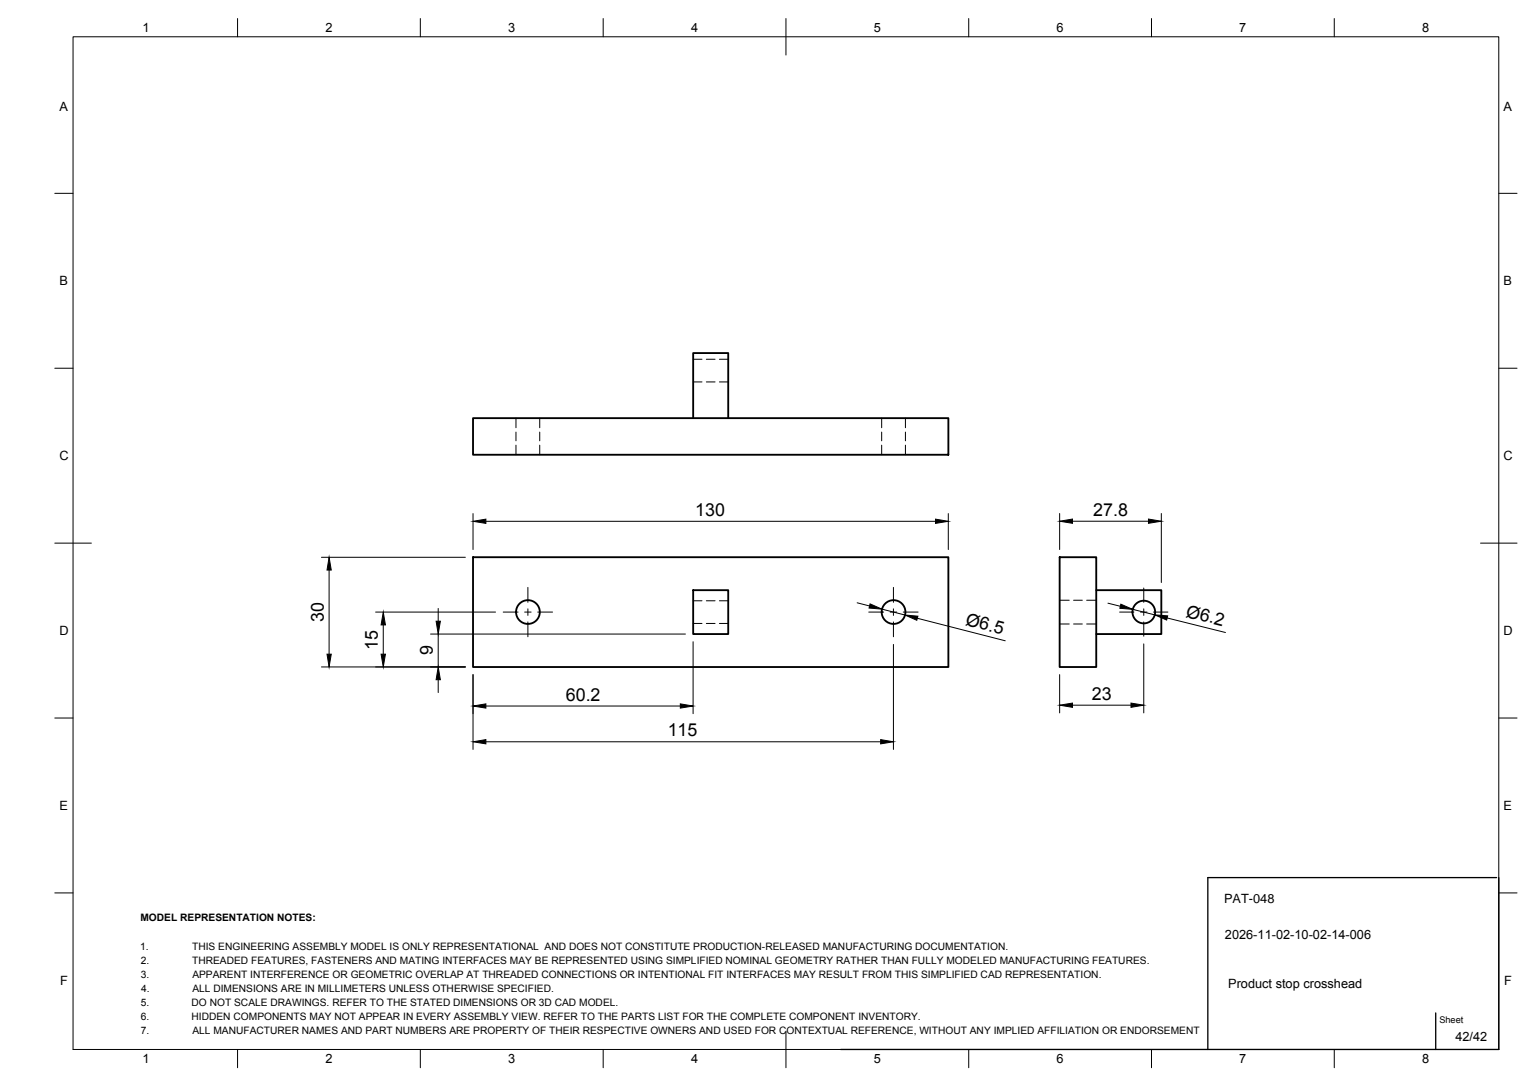
ISO-10303-21;
HEADER;
/* Generated by software containing ST-Developer
 * from STEP Tools, Inc. (www.steptools.com) 
 */

FILE_DESCRIPTION(
/* description */ ('Guided pneumatic stop gate'),
/* implementation_level */ '2;1');

FILE_NAME(
/* name */ 'Product stop crosshead.step',
/* time_stamp */ '2026-10-27T21:43:45-07:00',
/* author */ (''),
/* organization */ (''),
/* preprocessor_version */ 'ST-DEVELOPER v20.2',
/* originating_system */ 'Autodesk Translation Framework v15.17.0.0',
/* authorisation */ '');

FILE_SCHEMA (('AUTOMOTIVE_DESIGN { 1 0 10303 214 3 1 1 }'));
ENDSEC;

DATA;
#10=MECHANICAL_DESIGN_GEOMETRIC_PRESENTATION_REPRESENTATION('',(#574),#14392);
#490=SHAPE_REPRESENTATION_RELATIONSHIP('SRR','None',#14627,#532);
#532=ADVANCED_BREP_SHAPE_REPRESENTATION('',(#612),#14389);
#574=STYLED_ITEM('',(#14891),#612);
#612=MANIFOLD_SOLID_BREP('Body1',#7918);
#814=FACE_BOUND('',#2243,.T.);
#815=FACE_BOUND('',#2246,.T.);
#816=FACE_BOUND('',#2249,.T.);
#817=FACE_BOUND('',#2250,.T.);
#818=FACE_BOUND('',#2251,.T.);
#819=FACE_BOUND('',#2254,.T.);
#820=FACE_BOUND('',#2255,.T.);
#1097=PLANE('',#9325);
#1098=PLANE('',#9326);
#1099=PLANE('',#9327);
#1100=PLANE('',#9328);
#1101=PLANE('',#9329);
#1102=PLANE('',#9330);
#1103=PLANE('',#9331);
#1104=PLANE('',#9332);
#1105=PLANE('',#9333);
#1106=PLANE('',#9334);
#1107=PLANE('',#9335);
#1564=FACE_OUTER_BOUND('',#2238,.T.);
#1565=FACE_OUTER_BOUND('',#2239,.T.);
#1566=FACE_OUTER_BOUND('',#2240,.T.);
#1567=FACE_OUTER_BOUND('',#2241,.T.);
#1568=FACE_OUTER_BOUND('',#2242,.T.);
#1569=FACE_OUTER_BOUND('',#2244,.T.);
#1570=FACE_OUTER_BOUND('',#2245,.T.);
#1571=FACE_OUTER_BOUND('',#2247,.T.);
#1572=FACE_OUTER_BOUND('',#2248,.T.);
#1573=FACE_OUTER_BOUND('',#2252,.T.);
#1574=FACE_OUTER_BOUND('',#2253,.T.);
#1575=FACE_OUTER_BOUND('',#2256,.T.);
#1576=FACE_OUTER_BOUND('',#2257,.T.);
#1577=FACE_OUTER_BOUND('',#2258,.T.);
#2238=EDGE_LOOP('',(#7108,#7109,#7110,#7111));
#2239=EDGE_LOOP('',(#7112,#7113,#7114,#7115));
#2240=EDGE_LOOP('',(#7116,#7117,#7118,#7119));
#2241=EDGE_LOOP('',(#7120,#7121,#7122,#7123));
#2242=EDGE_LOOP('',(#7124,#7125,#7126,#7127));
#2243=EDGE_LOOP('',(#7128));
#2244=EDGE_LOOP('',(#7129,#7130,#7131,#7132));
#2245=EDGE_LOOP('',(#7133,#7134,#7135,#7136));
#2246=EDGE_LOOP('',(#7137));
#2247=EDGE_LOOP('',(#7138,#7139,#7140,#7141));
#2248=EDGE_LOOP('',(#7142,#7143,#7144,#7145));
#2249=EDGE_LOOP('',(#7146));
#2250=EDGE_LOOP('',(#7147));
#2251=EDGE_LOOP('',(#7148,#7149,#7150,#7151));
#2252=EDGE_LOOP('',(#7152,#7153,#7154,#7155));
#2253=EDGE_LOOP('',(#7156,#7157,#7158,#7159));
#2254=EDGE_LOOP('',(#7160));
#2255=EDGE_LOOP('',(#7161));
#2256=EDGE_LOOP('',(#7162,#7163,#7164,#7165));
#2257=EDGE_LOOP('',(#7166,#7167,#7168,#7169));
#2258=EDGE_LOOP('',(#7170,#7171,#7172,#7173));
#2785=LINE('',#14120,#3330);
#2786=LINE('',#14126,#3331);
#2787=LINE('',#14132,#3332);
#2788=LINE('',#14137,#3333);
#2789=LINE('',#14139,#3334);
#2790=LINE('',#14141,#3335);
#2791=LINE('',#14142,#3336);
#2792=LINE('',#14145,#3337);
#2793=LINE('',#14147,#3338);
#2794=LINE('',#14148,#3339);
#2795=LINE('',#14151,#3340);
#2796=LINE('',#14152,#3341);
#2797=LINE('',#14155,#3342);
#2798=LINE('',#14156,#3343);
#2799=LINE('',#14158,#3344);
#2800=LINE('',#14162,#3345);
#2801=LINE('',#14164,#3346);
#2802=LINE('',#14166,#3347);
#2803=LINE('',#14167,#3348);
#2804=LINE('',#14170,#3349);
#2805=LINE('',#14172,#3350);
#2806=LINE('',#14173,#3351);
#2807=LINE('',#14176,#3352);
#2808=LINE('',#14178,#3353);
#2809=LINE('',#14179,#3354);
#2810=LINE('',#14181,#3355);
#2811=LINE('',#14182,#3356);
#3330=VECTOR('',#11756,0.325);
#3331=VECTOR('',#11763,0.325);
#3332=VECTOR('',#11770,0.31);
#3333=VECTOR('',#11775,1.);
#3334=VECTOR('',#11776,1.);
#3335=VECTOR('',#11777,1.);
#3336=VECTOR('',#11778,1.);
#3337=VECTOR('',#11781,1.);
#3338=VECTOR('',#11782,1.);
#3339=VECTOR('',#11783,1.);
#3340=VECTOR('',#11786,1.);
#3341=VECTOR('',#11787,1.);
#3342=VECTOR('',#11790,1.);
#3343=VECTOR('',#11791,1.);
#3344=VECTOR('',#11794,1.);
#3345=VECTOR('',#11797,1.);
#3346=VECTOR('',#11798,1.);
#3347=VECTOR('',#11799,1.);
#3348=VECTOR('',#11800,1.);
#3349=VECTOR('',#11803,1.);
#3350=VECTOR('',#11804,1.);
#3351=VECTOR('',#11805,1.);
#3352=VECTOR('',#11808,1.);
#3353=VECTOR('',#11809,1.);
#3354=VECTOR('',#11810,1.);
#3355=VECTOR('',#11813,1.);
#3356=VECTOR('',#11814,1.);
#3723=CIRCLE('',#9317,0.325);
#3724=CIRCLE('',#9318,0.325);
#3725=CIRCLE('',#9320,0.325);
#3726=CIRCLE('',#9321,0.325);
#3727=CIRCLE('',#9323,0.31);
#3728=CIRCLE('',#9324,0.31);
#4314=VERTEX_POINT('',#14117);
#4315=VERTEX_POINT('',#14119);
#4316=VERTEX_POINT('',#14123);
#4317=VERTEX_POINT('',#14125);
#4318=VERTEX_POINT('',#14129);
#4319=VERTEX_POINT('',#14131);
#4320=VERTEX_POINT('',#14135);
#4321=VERTEX_POINT('',#14136);
#4322=VERTEX_POINT('',#14138);
#4323=VERTEX_POINT('',#14140);
#4324=VERTEX_POINT('',#14144);
#4325=VERTEX_POINT('',#14146);
#4326=VERTEX_POINT('',#14150);
#4327=VERTEX_POINT('',#14154);
#4328=VERTEX_POINT('',#14160);
#4329=VERTEX_POINT('',#14161);
#4330=VERTEX_POINT('',#14163);
#4331=VERTEX_POINT('',#14165);
#4332=VERTEX_POINT('',#14169);
#4333=VERTEX_POINT('',#14171);
#4334=VERTEX_POINT('',#14175);
#4335=VERTEX_POINT('',#14177);
#5252=EDGE_CURVE('',#4314,#4314,#3723,.T.);
#5253=EDGE_CURVE('',#4314,#4315,#2785,.T.);
#5254=EDGE_CURVE('',#4315,#4315,#3724,.T.);
#5255=EDGE_CURVE('',#4316,#4316,#3725,.T.);
#5256=EDGE_CURVE('',#4316,#4317,#2786,.T.);
#5257=EDGE_CURVE('',#4317,#4317,#3726,.T.);
#5258=EDGE_CURVE('',#4318,#4318,#3727,.T.);
#5259=EDGE_CURVE('',#4318,#4319,#2787,.T.);
#5260=EDGE_CURVE('',#4319,#4319,#3728,.T.);
#5261=EDGE_CURVE('',#4320,#4321,#2788,.T.);
#5262=EDGE_CURVE('',#4322,#4320,#2789,.T.);
#5263=EDGE_CURVE('',#4323,#4322,#2790,.T.);
#5264=EDGE_CURVE('',#4321,#4323,#2791,.T.);
#5265=EDGE_CURVE('',#4324,#4320,#2792,.T.);
#5266=EDGE_CURVE('',#4325,#4324,#2793,.T.);
#5267=EDGE_CURVE('',#4322,#4325,#2794,.T.);
#5268=EDGE_CURVE('',#4326,#4325,#2795,.T.);
#5269=EDGE_CURVE('',#4323,#4326,#2796,.T.);
#5270=EDGE_CURVE('',#4321,#4327,#2797,.T.);
#5271=EDGE_CURVE('',#4327,#4326,#2798,.T.);
#5272=EDGE_CURVE('',#4327,#4324,#2799,.T.);
#5273=EDGE_CURVE('',#4328,#4329,#2800,.T.);
#5274=EDGE_CURVE('',#4329,#4330,#2801,.T.);
#5275=EDGE_CURVE('',#4331,#4330,#2802,.T.);
#5276=EDGE_CURVE('',#4328,#4331,#2803,.T.);
#5277=EDGE_CURVE('',#4332,#4328,#2804,.T.);
#5278=EDGE_CURVE('',#4333,#4331,#2805,.T.);
#5279=EDGE_CURVE('',#4332,#4333,#2806,.T.);
#5280=EDGE_CURVE('',#4334,#4332,#2807,.T.);
#5281=EDGE_CURVE('',#4335,#4333,#2808,.T.);
#5282=EDGE_CURVE('',#4334,#4335,#2809,.T.);
#5283=EDGE_CURVE('',#4329,#4334,#2810,.T.);
#5284=EDGE_CURVE('',#4330,#4335,#2811,.T.);
#7108=ORIENTED_EDGE('',*,*,#5252,.F.);
#7109=ORIENTED_EDGE('',*,*,#5253,.T.);
#7110=ORIENTED_EDGE('',*,*,#5254,.F.);
#7111=ORIENTED_EDGE('',*,*,#5253,.F.);
#7112=ORIENTED_EDGE('',*,*,#5255,.F.);
#7113=ORIENTED_EDGE('',*,*,#5256,.T.);
#7114=ORIENTED_EDGE('',*,*,#5257,.F.);
#7115=ORIENTED_EDGE('',*,*,#5256,.F.);
#7116=ORIENTED_EDGE('',*,*,#5258,.F.);
#7117=ORIENTED_EDGE('',*,*,#5259,.T.);
#7118=ORIENTED_EDGE('',*,*,#5260,.F.);
#7119=ORIENTED_EDGE('',*,*,#5259,.F.);
#7120=ORIENTED_EDGE('',*,*,#5261,.F.);
#7121=ORIENTED_EDGE('',*,*,#5262,.F.);
#7122=ORIENTED_EDGE('',*,*,#5263,.F.);
#7123=ORIENTED_EDGE('',*,*,#5264,.F.);
#7124=ORIENTED_EDGE('',*,*,#5265,.F.);
#7125=ORIENTED_EDGE('',*,*,#5266,.F.);
#7126=ORIENTED_EDGE('',*,*,#5267,.F.);
#7127=ORIENTED_EDGE('',*,*,#5262,.T.);
#7128=ORIENTED_EDGE('',*,*,#5258,.T.);
#7129=ORIENTED_EDGE('',*,*,#5263,.T.);
#7130=ORIENTED_EDGE('',*,*,#5267,.T.);
#7131=ORIENTED_EDGE('',*,*,#5268,.F.);
#7132=ORIENTED_EDGE('',*,*,#5269,.F.);
#7133=ORIENTED_EDGE('',*,*,#5270,.F.);
#7134=ORIENTED_EDGE('',*,*,#5264,.T.);
#7135=ORIENTED_EDGE('',*,*,#5269,.T.);
#7136=ORIENTED_EDGE('',*,*,#5271,.F.);
#7137=ORIENTED_EDGE('',*,*,#5260,.T.);
#7138=ORIENTED_EDGE('',*,*,#5272,.F.);
#7139=ORIENTED_EDGE('',*,*,#5271,.T.);
#7140=ORIENTED_EDGE('',*,*,#5268,.T.);
#7141=ORIENTED_EDGE('',*,*,#5266,.T.);
#7142=ORIENTED_EDGE('',*,*,#5273,.T.);
#7143=ORIENTED_EDGE('',*,*,#5274,.T.);
#7144=ORIENTED_EDGE('',*,*,#5275,.F.);
#7145=ORIENTED_EDGE('',*,*,#5276,.F.);
#7146=ORIENTED_EDGE('',*,*,#5254,.T.);
#7147=ORIENTED_EDGE('',*,*,#5257,.T.);
#7148=ORIENTED_EDGE('',*,*,#5265,.T.);
#7149=ORIENTED_EDGE('',*,*,#5261,.T.);
#7150=ORIENTED_EDGE('',*,*,#5270,.T.);
#7151=ORIENTED_EDGE('',*,*,#5272,.T.);
#7152=ORIENTED_EDGE('',*,*,#5277,.T.);
#7153=ORIENTED_EDGE('',*,*,#5276,.T.);
#7154=ORIENTED_EDGE('',*,*,#5278,.F.);
#7155=ORIENTED_EDGE('',*,*,#5279,.F.);
#7156=ORIENTED_EDGE('',*,*,#5280,.T.);
#7157=ORIENTED_EDGE('',*,*,#5279,.T.);
#7158=ORIENTED_EDGE('',*,*,#5281,.F.);
#7159=ORIENTED_EDGE('',*,*,#5282,.F.);
#7160=ORIENTED_EDGE('',*,*,#5252,.T.);
#7161=ORIENTED_EDGE('',*,*,#5255,.T.);
#7162=ORIENTED_EDGE('',*,*,#5283,.T.);
#7163=ORIENTED_EDGE('',*,*,#5282,.T.);
#7164=ORIENTED_EDGE('',*,*,#5284,.F.);
#7165=ORIENTED_EDGE('',*,*,#5274,.F.);
#7166=ORIENTED_EDGE('',*,*,#5284,.T.);
#7167=ORIENTED_EDGE('',*,*,#5281,.T.);
#7168=ORIENTED_EDGE('',*,*,#5278,.T.);
#7169=ORIENTED_EDGE('',*,*,#5275,.T.);
#7170=ORIENTED_EDGE('',*,*,#5283,.F.);
#7171=ORIENTED_EDGE('',*,*,#5273,.F.);
#7172=ORIENTED_EDGE('',*,*,#5277,.F.);
#7173=ORIENTED_EDGE('',*,*,#5280,.F.);
#7394=CYLINDRICAL_SURFACE('',#9316,0.325);
#7395=CYLINDRICAL_SURFACE('',#9319,0.325);
#7396=CYLINDRICAL_SURFACE('',#9322,0.31);
#7846=ADVANCED_FACE('',(#1564),#7394,.F.);
#7847=ADVANCED_FACE('',(#1565),#7395,.F.);
#7848=ADVANCED_FACE('',(#1566),#7396,.F.);
#7849=ADVANCED_FACE('',(#1567),#1097,.F.);
#7850=ADVANCED_FACE('',(#1568,#814),#1098,.T.);
#7851=ADVANCED_FACE('',(#1569),#1099,.T.);
#7852=ADVANCED_FACE('',(#1570,#815),#1100,.T.);
#7853=ADVANCED_FACE('',(#1571),#1101,.T.);
#7854=ADVANCED_FACE('',(#1572,#816,#817,#818),#1102,.T.);
#7855=ADVANCED_FACE('',(#1573),#1103,.T.);
#7856=ADVANCED_FACE('',(#1574,#819,#820),#1104,.T.);
#7857=ADVANCED_FACE('',(#1575),#1105,.T.);
#7858=ADVANCED_FACE('',(#1576),#1106,.T.);
#7859=ADVANCED_FACE('',(#1577),#1107,.F.);
#7918=CLOSED_SHELL('',(#7846,#7847,#7848,#7849,#7850,#7851,#7852,#7853,
#7854,#7855,#7856,#7857,#7858,#7859));
#9315=AXIS2_PLACEMENT_3D('',#14115,#11750,#11751);
#9316=AXIS2_PLACEMENT_3D('',#14116,#11752,#11753);
#9317=AXIS2_PLACEMENT_3D('',#14118,#11754,#11755);
#9318=AXIS2_PLACEMENT_3D('',#14121,#11757,#11758);
#9319=AXIS2_PLACEMENT_3D('',#14122,#11759,#11760);
#9320=AXIS2_PLACEMENT_3D('',#14124,#11761,#11762);
#9321=AXIS2_PLACEMENT_3D('',#14127,#11764,#11765);
#9322=AXIS2_PLACEMENT_3D('',#14128,#11766,#11767);
#9323=AXIS2_PLACEMENT_3D('',#14130,#11768,#11769);
#9324=AXIS2_PLACEMENT_3D('',#14133,#11771,#11772);
#9325=AXIS2_PLACEMENT_3D('',#14134,#11773,#11774);
#9326=AXIS2_PLACEMENT_3D('',#14143,#11779,#11780);
#9327=AXIS2_PLACEMENT_3D('',#14149,#11784,#11785);
#9328=AXIS2_PLACEMENT_3D('',#14153,#11788,#11789);
#9329=AXIS2_PLACEMENT_3D('',#14157,#11792,#11793);
#9330=AXIS2_PLACEMENT_3D('',#14159,#11795,#11796);
#9331=AXIS2_PLACEMENT_3D('',#14168,#11801,#11802);
#9332=AXIS2_PLACEMENT_3D('',#14174,#11806,#11807);
#9333=AXIS2_PLACEMENT_3D('',#14180,#11811,#11812);
#9334=AXIS2_PLACEMENT_3D('',#14183,#11815,#11816);
#9335=AXIS2_PLACEMENT_3D('',#14184,#11817,#11818);
#11750=DIRECTION('axis',(0.,0.,1.));
#11751=DIRECTION('refdir',(1.,0.,0.));
#11752=DIRECTION('center_axis',(0.,1.,0.));
#11753=DIRECTION('ref_axis',(1.,0.,0.));
#11754=DIRECTION('center_axis',(0.,1.,0.));
#11755=DIRECTION('ref_axis',(1.,0.,0.));
#11756=DIRECTION('',(0.,1.,0.));
#11757=DIRECTION('center_axis',(0.,-1.,0.));
#11758=DIRECTION('ref_axis',(1.,0.,0.));
#11759=DIRECTION('center_axis',(0.,1.,0.));
#11760=DIRECTION('ref_axis',(1.,0.,0.));
#11761=DIRECTION('center_axis',(0.,1.,0.));
#11762=DIRECTION('ref_axis',(1.,0.,0.));
#11763=DIRECTION('',(0.,1.,0.));
#11764=DIRECTION('center_axis',(0.,-1.,0.));
#11765=DIRECTION('ref_axis',(1.,0.,0.));
#11766=DIRECTION('center_axis',(1.,0.,0.));
#11767=DIRECTION('ref_axis',(0.,0.,-1.));
#11768=DIRECTION('center_axis',(1.,0.,0.));
#11769=DIRECTION('ref_axis',(0.,0.,-1.));
#11770=DIRECTION('',(1.,0.,0.));
#11771=DIRECTION('center_axis',(-1.,0.,0.));
#11772=DIRECTION('ref_axis',(0.,0.,-1.));
#11773=DIRECTION('center_axis',(0.,0.,1.));
#11774=DIRECTION('ref_axis',(1.,0.,0.));
#11775=DIRECTION('',(1.,0.,0.));
#11776=DIRECTION('',(0.,-1.,0.));
#11777=DIRECTION('',(-1.,0.,0.));
#11778=DIRECTION('',(0.,1.,0.));
#11779=DIRECTION('center_axis',(-1.,0.,0.));
#11780=DIRECTION('ref_axis',(0.,-1.,0.));
#11781=DIRECTION('',(0.,0.,-1.));
#11782=DIRECTION('',(0.,-1.,0.));
#11783=DIRECTION('',(0.,0.,1.));
#11784=DIRECTION('center_axis',(0.,1.,0.));
#11785=DIRECTION('ref_axis',(-1.,0.,0.));
#11786=DIRECTION('',(-1.,0.,0.));
#11787=DIRECTION('',(0.,0.,1.));
#11788=DIRECTION('center_axis',(1.,0.,0.));
#11789=DIRECTION('ref_axis',(0.,1.,0.));
#11790=DIRECTION('',(0.,0.,1.));
#11791=DIRECTION('',(0.,1.,0.));
#11792=DIRECTION('center_axis',(0.,0.,1.));
#11793=DIRECTION('ref_axis',(1.,0.,0.));
#11794=DIRECTION('',(-1.,0.,0.));
#11795=DIRECTION('center_axis',(0.,1.,0.));
#11796=DIRECTION('ref_axis',(-1.,0.,0.));
#11797=DIRECTION('',(-1.,0.,0.));
#11798=DIRECTION('',(0.,0.,1.));
#11799=DIRECTION('',(-1.,0.,0.));
#11800=DIRECTION('',(0.,0.,1.));
#11801=DIRECTION('center_axis',(1.,0.,0.));
#11802=DIRECTION('ref_axis',(0.,1.,0.));
#11803=DIRECTION('',(0.,1.,0.));
#11804=DIRECTION('',(0.,1.,0.));
#11805=DIRECTION('',(0.,0.,1.));
#11806=DIRECTION('center_axis',(0.,-1.,0.));
#11807=DIRECTION('ref_axis',(1.,0.,0.));
#11808=DIRECTION('',(1.,0.,0.));
#11809=DIRECTION('',(1.,0.,0.));
#11810=DIRECTION('',(0.,0.,1.));
#11811=DIRECTION('center_axis',(-1.,0.,0.));
#11812=DIRECTION('ref_axis',(0.,-1.,0.));
#11813=DIRECTION('',(0.,-1.,0.));
#11814=DIRECTION('',(0.,-1.,0.));
#11815=DIRECTION('center_axis',(0.,0.,1.));
#11816=DIRECTION('ref_axis',(1.,0.,0.));
#11817=DIRECTION('center_axis',(0.,0.,1.));
#11818=DIRECTION('ref_axis',(1.,0.,0.));
#14115=CARTESIAN_POINT('',(0.,0.,0.));
#14116=CARTESIAN_POINT('Origin',(-5.,-8.5,4.5));
#14117=CARTESIAN_POINT('',(-5.325,-8.4,4.5));
#14118=CARTESIAN_POINT('Origin',(-5.,-8.4,4.5));
#14119=CARTESIAN_POINT('',(-5.325,-7.4,4.5));
#14120=CARTESIAN_POINT('',(-5.325,-8.5,4.5));
#14121=CARTESIAN_POINT('Origin',(-5.,-7.4,4.5));
#14122=CARTESIAN_POINT('Origin',(5.,-8.5,4.5));
#14123=CARTESIAN_POINT('',(4.675,-8.4,4.5));
#14124=CARTESIAN_POINT('Origin',(5.,-8.4,4.5));
#14125=CARTESIAN_POINT('',(4.675,-7.4,4.5));
#14126=CARTESIAN_POINT('',(4.675,-8.5,4.5));
#14127=CARTESIAN_POINT('Origin',(5.,-7.4,4.5));
#14128=CARTESIAN_POINT('Origin',(-0.6,-6.1,4.5));
#14129=CARTESIAN_POINT('',(-0.48,-6.1,4.81));
#14130=CARTESIAN_POINT('Origin',(-0.48,-6.1,4.5));
#14131=CARTESIAN_POINT('',(0.48,-6.1,4.81));
#14132=CARTESIAN_POINT('',(-0.6,-6.1,4.81));
#14133=CARTESIAN_POINT('Origin',(0.48,-6.1,4.5));
#14134=CARTESIAN_POINT('Origin',(0.,-7.01,3.9));
#14135=CARTESIAN_POINT('',(-0.48,-7.4,3.9));
#14136=CARTESIAN_POINT('',(0.48,-7.4,3.9));
#14137=CARTESIAN_POINT('',(3.25,-7.4,3.9));
#14138=CARTESIAN_POINT('',(-0.48,-5.62,3.9));
#14139=CARTESIAN_POINT('',(-0.48,-5.62,3.9));
#14140=CARTESIAN_POINT('',(0.48,-5.62,3.9));
#14141=CARTESIAN_POINT('',(0.48,-5.62,3.9));
#14142=CARTESIAN_POINT('',(0.48,-8.4,3.9));
#14143=CARTESIAN_POINT('Origin',(-0.48,-5.62,3.9));
#14144=CARTESIAN_POINT('',(-0.48,-7.4,5.1));
#14145=CARTESIAN_POINT('',(-0.48,-7.4,3.45));
#14146=CARTESIAN_POINT('',(-0.48,-5.62,5.1));
#14147=CARTESIAN_POINT('',(-0.48,-5.62,5.1));
#14148=CARTESIAN_POINT('',(-0.48,-5.62,3.9));
#14149=CARTESIAN_POINT('Origin',(0.48,-5.62,3.9));
#14150=CARTESIAN_POINT('',(0.48,-5.62,5.1));
#14151=CARTESIAN_POINT('',(0.48,-5.62,5.1));
#14152=CARTESIAN_POINT('',(0.48,-5.62,3.9));
#14153=CARTESIAN_POINT('Origin',(0.48,-8.4,3.9));
#14154=CARTESIAN_POINT('',(0.48,-7.4,5.1));
#14155=CARTESIAN_POINT('',(0.48,-7.4,3.45));
#14156=CARTESIAN_POINT('',(0.48,-8.4,5.1));
#14157=CARTESIAN_POINT('Origin',(0.,-7.01,5.1));
#14158=CARTESIAN_POINT('',(3.25,-7.4,5.1));
#14159=CARTESIAN_POINT('Origin',(6.5,-7.4,3.));
#14160=CARTESIAN_POINT('',(6.5,-7.4,3.));
#14161=CARTESIAN_POINT('',(-6.5,-7.4,3.));
#14162=CARTESIAN_POINT('',(6.5,-7.4,3.));
#14163=CARTESIAN_POINT('',(-6.5,-7.4,6.));
#14164=CARTESIAN_POINT('',(-6.5,-7.4,3.));
#14165=CARTESIAN_POINT('',(6.5,-7.4,6.));
#14166=CARTESIAN_POINT('',(6.5,-7.4,6.));
#14167=CARTESIAN_POINT('',(6.5,-7.4,3.));
#14168=CARTESIAN_POINT('Origin',(6.5,-8.4,3.));
#14169=CARTESIAN_POINT('',(6.5,-8.4,3.));
#14170=CARTESIAN_POINT('',(6.5,-8.4,3.));
#14171=CARTESIAN_POINT('',(6.5,-8.4,6.));
#14172=CARTESIAN_POINT('',(6.5,-8.4,6.));
#14173=CARTESIAN_POINT('',(6.5,-8.4,3.));
#14174=CARTESIAN_POINT('Origin',(-6.5,-8.4,3.));
#14175=CARTESIAN_POINT('',(-6.5,-8.4,3.));
#14176=CARTESIAN_POINT('',(-6.5,-8.4,3.));
#14177=CARTESIAN_POINT('',(-6.5,-8.4,6.));
#14178=CARTESIAN_POINT('',(-6.5,-8.4,6.));
#14179=CARTESIAN_POINT('',(-6.5,-8.4,3.));
#14180=CARTESIAN_POINT('Origin',(-6.5,-7.4,3.));
#14181=CARTESIAN_POINT('',(-6.5,-7.4,3.));
#14182=CARTESIAN_POINT('',(-6.5,-7.4,6.));
#14183=CARTESIAN_POINT('Origin',(0.,-7.9,6.));
#14184=CARTESIAN_POINT('Origin',(0.,-7.9,3.));
#14341=UNCERTAINTY_MEASURE_WITH_UNIT(LENGTH_MEASURE(0.001),#14393,
'DISTANCE_ACCURACY_VALUE',
'Maximum model space distance between geometric entities at asserted c
onnectivities');
#14344=UNCERTAINTY_MEASURE_WITH_UNIT(LENGTH_MEASURE(0.001),#14393,
'DISTANCE_ACCURACY_VALUE',
'Maximum model space distance between geometric entities at asserted c
onnectivities');
#14389=(
GEOMETRIC_REPRESENTATION_CONTEXT(3)
GLOBAL_UNCERTAINTY_ASSIGNED_CONTEXT((#14341))
GLOBAL_UNIT_ASSIGNED_CONTEXT((#14393,#14395,#14396))
REPRESENTATION_CONTEXT('','3D')
);
#14392=(
GEOMETRIC_REPRESENTATION_CONTEXT(3)
GLOBAL_UNCERTAINTY_ASSIGNED_CONTEXT((#14344))
GLOBAL_UNIT_ASSIGNED_CONTEXT((#14393,#14395,#14396))
REPRESENTATION_CONTEXT('','3D')
);
#14393=(
LENGTH_UNIT()
NAMED_UNIT(*)
SI_UNIT(.CENTI.,.METRE.)
);
#14395=(
NAMED_UNIT(*)
PLANE_ANGLE_UNIT()
SI_UNIT($,.RADIAN.)
);
#14396=(
NAMED_UNIT(*)
SI_UNIT($,.STERADIAN.)
SOLID_ANGLE_UNIT()
);
#14441=SHAPE_DEFINITION_REPRESENTATION(#14560,#14627);
#14560=PRODUCT_DEFINITION_SHAPE('',$,#14675);
#14627=SHAPE_REPRESENTATION('',(#9315),#14389);
#14630=PRODUCT_DEFINITION_CONTEXT('part definition',#14773,'design');
#14675=PRODUCT_DEFINITION('Product stop crosshead',
'Product stop crosshead',#14722,#14630);
#14722=PRODUCT_DEFINITION_FORMATION('',$,#14819);
#14773=APPLICATION_CONTEXT(
'Core Data for Automotive Mechanical Design Process');
#14774=PRODUCT_CONTEXT('part definition',#14773,'mechanical');
#14819=PRODUCT('Product stop crosshead','Product stop crosshead',
'Product stop crosshead',(#14774));
#14885=COLOUR_RGB('Grey',0.48,0.52,0.57);
#14886=FILL_AREA_STYLE_COLOUR('',#14885);
#14887=FILL_AREA_STYLE('',(#14886));
#14888=SURFACE_STYLE_FILL_AREA(#14887);
#14889=SURFACE_SIDE_STYLE('',(#14888));
#14890=SURFACE_STYLE_USAGE(.BOTH.,#14889);
#14891=PRESENTATION_STYLE_ASSIGNMENT((#14890));
ENDSEC;
END-ISO-10303-21;
